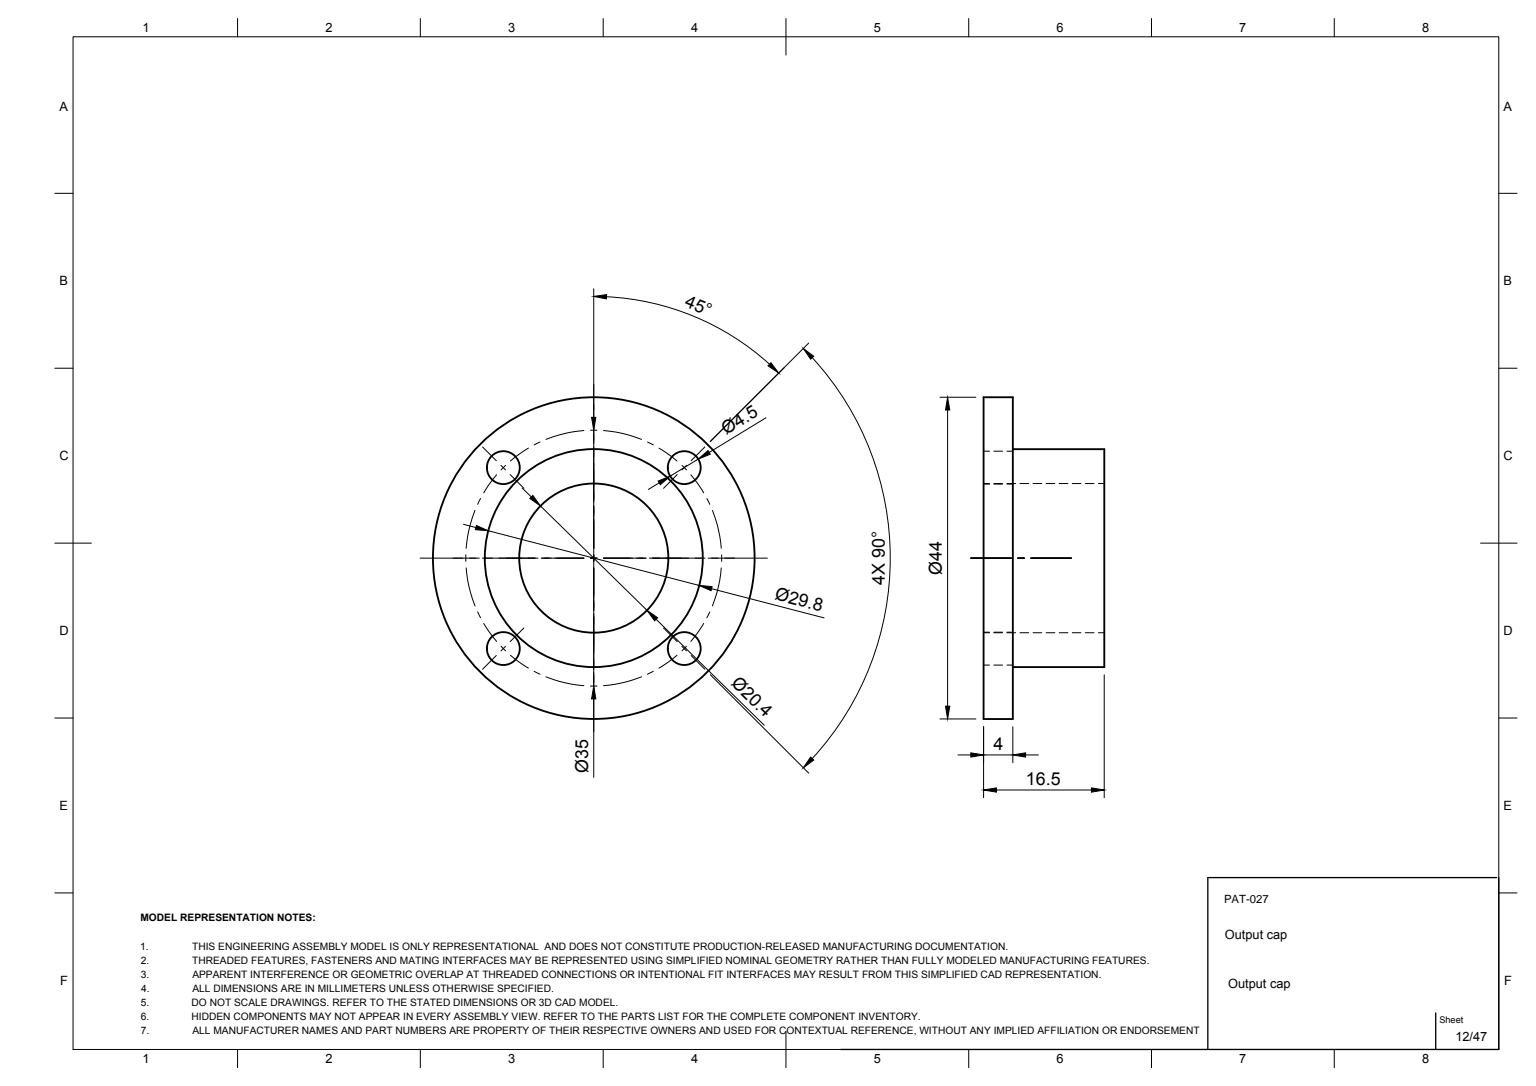
ISO-10303-21;
HEADER;
/* Generated by software containing ST-Developer
 * from STEP Tools, Inc. (www.steptools.com) 
 */

FILE_DESCRIPTION(
/* description */ ('Crank-driven oscillating fan base (mechanism only)'),

/* implementation_level */ '2;1');

FILE_NAME(
/* name */ 'Output cap.step',
/* time_stamp */ '2026-10-28T03:25:00-07:00',
/* author */ (''),
/* organization */ (''),
/* preprocessor_version */ 'ST-DEVELOPER v20.2',
/* originating_system */ 'Autodesk Translation Framework v15.17.0.0',
/* authorisation */ '');

FILE_SCHEMA (('AUTOMOTIVE_DESIGN { 1 0 10303 214 3 1 1 }'));
ENDSEC;

DATA;
#10=MECHANICAL_DESIGN_GEOMETRIC_PRESENTATION_REPRESENTATION('',(#444),#11916);
#364=SHAPE_REPRESENTATION_RELATIONSHIP('SRR','None',#12088,#404);
#404=ADVANCED_BREP_SHAPE_REPRESENTATION('',(#492),#11879);
#444=STYLED_ITEM('',(#12361),#492);
#492=MANIFOLD_SOLID_BREP('Body1',#6074);
#595=FACE_BOUND('',#1430,.T.);
#596=FACE_BOUND('',#1434,.T.);
#597=FACE_BOUND('',#1435,.T.);
#598=FACE_BOUND('',#1436,.T.);
#599=FACE_BOUND('',#1437,.T.);
#600=FACE_BOUND('',#1438,.T.);
#601=FACE_BOUND('',#1440,.T.);
#602=FACE_BOUND('',#1441,.T.);
#603=FACE_BOUND('',#1442,.T.);
#604=FACE_BOUND('',#1443,.T.);
#605=FACE_BOUND('',#1444,.T.);
#739=PLANE('',#6796);
#740=PLANE('',#6803);
#741=PLANE('',#6804);
#984=FACE_OUTER_BOUND('',#1424,.T.);
#985=FACE_OUTER_BOUND('',#1425,.T.);
#986=FACE_OUTER_BOUND('',#1426,.T.);
#987=FACE_OUTER_BOUND('',#1427,.T.);
#988=FACE_OUTER_BOUND('',#1428,.T.);
#989=FACE_OUTER_BOUND('',#1429,.T.);
#990=FACE_OUTER_BOUND('',#1431,.T.);
#991=FACE_OUTER_BOUND('',#1432,.T.);
#992=FACE_OUTER_BOUND('',#1433,.T.);
#993=FACE_OUTER_BOUND('',#1439,.T.);
#1424=EDGE_LOOP('',(#4502,#4503,#4504,#4505));
#1425=EDGE_LOOP('',(#4506,#4507,#4508,#4509));
#1426=EDGE_LOOP('',(#4510,#4511,#4512,#4513));
#1427=EDGE_LOOP('',(#4514,#4515,#4516,#4517));
#1428=EDGE_LOOP('',(#4518,#4519,#4520,#4521));
#1429=EDGE_LOOP('',(#4522));
#1430=EDGE_LOOP('',(#4523));
#1431=EDGE_LOOP('',(#4524,#4525,#4526,#4527));
#1432=EDGE_LOOP('',(#4528,#4529,#4530,#4531));
#1433=EDGE_LOOP('',(#4532));
#1434=EDGE_LOOP('',(#4533));
#1435=EDGE_LOOP('',(#4534));
#1436=EDGE_LOOP('',(#4535));
#1437=EDGE_LOOP('',(#4536));
#1438=EDGE_LOOP('',(#4537));
#1439=EDGE_LOOP('',(#4538));
#1440=EDGE_LOOP('',(#4539));
#1441=EDGE_LOOP('',(#4540));
#1442=EDGE_LOOP('',(#4541));
#1443=EDGE_LOOP('',(#4542));
#1444=EDGE_LOOP('',(#4543));
#1893=LINE('',#10059,#2226);
#1894=LINE('',#10065,#2227);
#1895=LINE('',#10071,#2228);
#1896=LINE('',#10077,#2229);
#1897=LINE('',#10083,#2230);
#1898=LINE('',#10091,#2231);
#1899=LINE('',#10096,#2232);
#2226=VECTOR('',#7954,0.225);
#2227=VECTOR('',#7961,0.225);
#2228=VECTOR('',#7968,0.225);
#2229=VECTOR('',#7975,0.225);
#2230=VECTOR('',#7982,1.49);
#2231=VECTOR('',#7993,1.02);
#2232=VECTOR('',#7998,2.2);
#2578=CIRCLE('',#6782,0.225);
#2579=CIRCLE('',#6783,0.225);
#2580=CIRCLE('',#6785,0.225);
#2581=CIRCLE('',#6786,0.225);
#2582=CIRCLE('',#6788,0.225);
#2583=CIRCLE('',#6789,0.225);
#2584=CIRCLE('',#6791,0.225);
#2585=CIRCLE('',#6792,0.225);
#2586=CIRCLE('',#6794,1.49);
#2587=CIRCLE('',#6795,1.49);
#2588=CIRCLE('',#6797,1.02);
#2589=CIRCLE('',#6799,1.02);
#2590=CIRCLE('',#6801,2.2);
#2591=CIRCLE('',#6802,2.2);
#2975=VERTEX_POINT('',#10056);
#2976=VERTEX_POINT('',#10058);
#2977=VERTEX_POINT('',#10062);
#2978=VERTEX_POINT('',#10064);
#2979=VERTEX_POINT('',#10068);
#2980=VERTEX_POINT('',#10070);
#2981=VERTEX_POINT('',#10074);
#2982=VERTEX_POINT('',#10076);
#2983=VERTEX_POINT('',#10080);
#2984=VERTEX_POINT('',#10082);
#2985=VERTEX_POINT('',#10086);
#2986=VERTEX_POINT('',#10089);
#2987=VERTEX_POINT('',#10093);
#2988=VERTEX_POINT('',#10095);
#3546=EDGE_CURVE('',#2975,#2975,#2578,.T.);
#3547=EDGE_CURVE('',#2975,#2976,#1893,.T.);
#3548=EDGE_CURVE('',#2976,#2976,#2579,.T.);
#3549=EDGE_CURVE('',#2977,#2977,#2580,.T.);
#3550=EDGE_CURVE('',#2977,#2978,#1894,.T.);
#3551=EDGE_CURVE('',#2978,#2978,#2581,.T.);
#3552=EDGE_CURVE('',#2979,#2979,#2582,.T.);
#3553=EDGE_CURVE('',#2979,#2980,#1895,.T.);
#3554=EDGE_CURVE('',#2980,#2980,#2583,.T.);
#3555=EDGE_CURVE('',#2981,#2981,#2584,.T.);
#3556=EDGE_CURVE('',#2981,#2982,#1896,.T.);
#3557=EDGE_CURVE('',#2982,#2982,#2585,.T.);
#3558=EDGE_CURVE('',#2983,#2983,#2586,.T.);
#3559=EDGE_CURVE('',#2983,#2984,#1897,.T.);
#3560=EDGE_CURVE('',#2984,#2984,#2587,.T.);
#3561=EDGE_CURVE('',#2985,#2985,#2588,.T.);
#3562=EDGE_CURVE('',#2986,#2986,#2589,.T.);
#3563=EDGE_CURVE('',#2986,#2985,#1898,.T.);
#3564=EDGE_CURVE('',#2987,#2987,#2590,.T.);
#3565=EDGE_CURVE('',#2987,#2988,#1899,.T.);
#3566=EDGE_CURVE('',#2988,#2988,#2591,.T.);
#4502=ORIENTED_EDGE('',*,*,#3546,.F.);
#4503=ORIENTED_EDGE('',*,*,#3547,.T.);
#4504=ORIENTED_EDGE('',*,*,#3548,.F.);
#4505=ORIENTED_EDGE('',*,*,#3547,.F.);
#4506=ORIENTED_EDGE('',*,*,#3549,.F.);
#4507=ORIENTED_EDGE('',*,*,#3550,.T.);
#4508=ORIENTED_EDGE('',*,*,#3551,.F.);
#4509=ORIENTED_EDGE('',*,*,#3550,.F.);
#4510=ORIENTED_EDGE('',*,*,#3552,.F.);
#4511=ORIENTED_EDGE('',*,*,#3553,.T.);
#4512=ORIENTED_EDGE('',*,*,#3554,.F.);
#4513=ORIENTED_EDGE('',*,*,#3553,.F.);
#4514=ORIENTED_EDGE('',*,*,#3555,.F.);
#4515=ORIENTED_EDGE('',*,*,#3556,.T.);
#4516=ORIENTED_EDGE('',*,*,#3557,.F.);
#4517=ORIENTED_EDGE('',*,*,#3556,.F.);
#4518=ORIENTED_EDGE('',*,*,#3558,.F.);
#4519=ORIENTED_EDGE('',*,*,#3559,.T.);
#4520=ORIENTED_EDGE('',*,*,#3560,.T.);
#4521=ORIENTED_EDGE('',*,*,#3559,.F.);
#4522=ORIENTED_EDGE('',*,*,#3560,.F.);
#4523=ORIENTED_EDGE('',*,*,#3561,.F.);
#4524=ORIENTED_EDGE('',*,*,#3562,.F.);
#4525=ORIENTED_EDGE('',*,*,#3563,.T.);
#4526=ORIENTED_EDGE('',*,*,#3561,.T.);
#4527=ORIENTED_EDGE('',*,*,#3563,.F.);
#4528=ORIENTED_EDGE('',*,*,#3564,.F.);
#4529=ORIENTED_EDGE('',*,*,#3565,.T.);
#4530=ORIENTED_EDGE('',*,*,#3566,.T.);
#4531=ORIENTED_EDGE('',*,*,#3565,.F.);
#4532=ORIENTED_EDGE('',*,*,#3564,.T.);
#4533=ORIENTED_EDGE('',*,*,#3562,.T.);
#4534=ORIENTED_EDGE('',*,*,#3557,.T.);
#4535=ORIENTED_EDGE('',*,*,#3554,.T.);
#4536=ORIENTED_EDGE('',*,*,#3551,.T.);
#4537=ORIENTED_EDGE('',*,*,#3548,.T.);
#4538=ORIENTED_EDGE('',*,*,#3566,.F.);
#4539=ORIENTED_EDGE('',*,*,#3558,.T.);
#4540=ORIENTED_EDGE('',*,*,#3555,.T.);
#4541=ORIENTED_EDGE('',*,*,#3552,.T.);
#4542=ORIENTED_EDGE('',*,*,#3549,.T.);
#4543=ORIENTED_EDGE('',*,*,#3546,.T.);
#5597=CYLINDRICAL_SURFACE('',#6781,0.225);
#5598=CYLINDRICAL_SURFACE('',#6784,0.225);
#5599=CYLINDRICAL_SURFACE('',#6787,0.225);
#5600=CYLINDRICAL_SURFACE('',#6790,0.225);
#5601=CYLINDRICAL_SURFACE('',#6793,1.49);
#5602=CYLINDRICAL_SURFACE('',#6798,1.02);
#5603=CYLINDRICAL_SURFACE('',#6800,2.2);
#5790=ADVANCED_FACE('',(#984),#5597,.F.);
#5791=ADVANCED_FACE('',(#985),#5598,.F.);
#5792=ADVANCED_FACE('',(#986),#5599,.F.);
#5793=ADVANCED_FACE('',(#987),#5600,.F.);
#5794=ADVANCED_FACE('',(#988),#5601,.T.);
#5795=ADVANCED_FACE('',(#989,#595),#739,.F.);
#5796=ADVANCED_FACE('',(#990),#5602,.F.);
#5797=ADVANCED_FACE('',(#991),#5603,.T.);
#5798=ADVANCED_FACE('',(#992,#596,#597,#598,#599,#600),#740,.T.);
#5799=ADVANCED_FACE('',(#993,#601,#602,#603,#604,#605),#741,.F.);
#6074=CLOSED_SHELL('',(#5790,#5791,#5792,#5793,#5794,#5795,#5796,#5797,
#5798,#5799));
#6780=AXIS2_PLACEMENT_3D('',#10054,#7948,#7949);
#6781=AXIS2_PLACEMENT_3D('',#10055,#7950,#7951);
#6782=AXIS2_PLACEMENT_3D('',#10057,#7952,#7953);
#6783=AXIS2_PLACEMENT_3D('',#10060,#7955,#7956);
#6784=AXIS2_PLACEMENT_3D('',#10061,#7957,#7958);
#6785=AXIS2_PLACEMENT_3D('',#10063,#7959,#7960);
#6786=AXIS2_PLACEMENT_3D('',#10066,#7962,#7963);
#6787=AXIS2_PLACEMENT_3D('',#10067,#7964,#7965);
#6788=AXIS2_PLACEMENT_3D('',#10069,#7966,#7967);
#6789=AXIS2_PLACEMENT_3D('',#10072,#7969,#7970);
#6790=AXIS2_PLACEMENT_3D('',#10073,#7971,#7972);
#6791=AXIS2_PLACEMENT_3D('',#10075,#7973,#7974);
#6792=AXIS2_PLACEMENT_3D('',#10078,#7976,#7977);
#6793=AXIS2_PLACEMENT_3D('',#10079,#7978,#7979);
#6794=AXIS2_PLACEMENT_3D('',#10081,#7980,#7981);
#6795=AXIS2_PLACEMENT_3D('',#10084,#7983,#7984);
#6796=AXIS2_PLACEMENT_3D('',#10085,#7985,#7986);
#6797=AXIS2_PLACEMENT_3D('',#10087,#7987,#7988);
#6798=AXIS2_PLACEMENT_3D('',#10088,#7989,#7990);
#6799=AXIS2_PLACEMENT_3D('',#10090,#7991,#7992);
#6800=AXIS2_PLACEMENT_3D('',#10092,#7994,#7995);
#6801=AXIS2_PLACEMENT_3D('',#10094,#7996,#7997);
#6802=AXIS2_PLACEMENT_3D('',#10097,#7999,#8000);
#6803=AXIS2_PLACEMENT_3D('',#10098,#8001,#8002);
#6804=AXIS2_PLACEMENT_3D('',#10099,#8003,#8004);
#7948=DIRECTION('axis',(0.,0.,1.));
#7949=DIRECTION('refdir',(1.,0.,0.));
#7950=DIRECTION('center_axis',(0.,0.,1.));
#7951=DIRECTION('ref_axis',(1.,0.,0.));
#7952=DIRECTION('center_axis',(0.,0.,1.));
#7953=DIRECTION('ref_axis',(1.,0.,0.));
#7954=DIRECTION('',(0.,0.,1.));
#7955=DIRECTION('center_axis',(0.,0.,-1.));
#7956=DIRECTION('ref_axis',(1.,0.,0.));
#7957=DIRECTION('center_axis',(0.,0.,1.));
#7958=DIRECTION('ref_axis',(1.,0.,0.));
#7959=DIRECTION('center_axis',(0.,0.,1.));
#7960=DIRECTION('ref_axis',(1.,0.,0.));
#7961=DIRECTION('',(0.,0.,1.));
#7962=DIRECTION('center_axis',(0.,0.,-1.));
#7963=DIRECTION('ref_axis',(1.,0.,0.));
#7964=DIRECTION('center_axis',(0.,0.,1.));
#7965=DIRECTION('ref_axis',(1.,0.,0.));
#7966=DIRECTION('center_axis',(0.,0.,1.));
#7967=DIRECTION('ref_axis',(1.,0.,0.));
#7968=DIRECTION('',(0.,0.,1.));
#7969=DIRECTION('center_axis',(0.,0.,-1.));
#7970=DIRECTION('ref_axis',(1.,0.,0.));
#7971=DIRECTION('center_axis',(0.,0.,1.));
#7972=DIRECTION('ref_axis',(1.,0.,0.));
#7973=DIRECTION('center_axis',(0.,0.,1.));
#7974=DIRECTION('ref_axis',(1.,0.,0.));
#7975=DIRECTION('',(0.,0.,1.));
#7976=DIRECTION('center_axis',(0.,0.,-1.));
#7977=DIRECTION('ref_axis',(1.,0.,0.));
#7978=DIRECTION('center_axis',(0.,0.,1.));
#7979=DIRECTION('ref_axis',(1.,0.,0.));
#7980=DIRECTION('center_axis',(0.,0.,1.));
#7981=DIRECTION('ref_axis',(1.,0.,0.));
#7982=DIRECTION('',(0.,0.,-1.));
#7983=DIRECTION('center_axis',(0.,0.,1.));
#7984=DIRECTION('ref_axis',(1.,0.,0.));
#7985=DIRECTION('center_axis',(0.,0.,1.));
#7986=DIRECTION('ref_axis',(1.,0.,0.));
#7987=DIRECTION('center_axis',(0.,0.,-1.));
#7988=DIRECTION('ref_axis',(1.,0.,0.));
#7989=DIRECTION('center_axis',(0.,0.,1.));
#7990=DIRECTION('ref_axis',(1.,0.,0.));
#7991=DIRECTION('center_axis',(0.,0.,-1.));
#7992=DIRECTION('ref_axis',(1.,0.,0.));
#7993=DIRECTION('',(0.,0.,-1.));
#7994=DIRECTION('center_axis',(0.,0.,1.));
#7995=DIRECTION('ref_axis',(1.,0.,0.));
#7996=DIRECTION('center_axis',(0.,0.,1.));
#7997=DIRECTION('ref_axis',(1.,0.,0.));
#7998=DIRECTION('',(0.,0.,-1.));
#7999=DIRECTION('center_axis',(0.,0.,1.));
#8000=DIRECTION('ref_axis',(1.,0.,0.));
#8001=DIRECTION('center_axis',(0.,0.,1.));
#8002=DIRECTION('ref_axis',(1.,0.,0.));
#8003=DIRECTION('center_axis',(0.,0.,1.));
#8004=DIRECTION('ref_axis',(1.,0.,0.));
#10054=CARTESIAN_POINT('',(0.,0.,0.));
#10055=CARTESIAN_POINT('Origin',(6.76256313292354,-1.23743686707646,5.1));
#10056=CARTESIAN_POINT('',(6.53756313292354,-1.23743686707646,5.2));
#10057=CARTESIAN_POINT('Origin',(6.76256313292354,-1.23743686707646,5.2));
#10058=CARTESIAN_POINT('',(6.53756313292354,-1.23743686707646,5.6));
#10059=CARTESIAN_POINT('',(6.53756313292354,-1.23743686707646,5.1));
#10060=CARTESIAN_POINT('Origin',(6.76256313292354,-1.23743686707646,5.6));
#10061=CARTESIAN_POINT('Origin',(6.76256313292354,1.23743686707646,5.1));
#10062=CARTESIAN_POINT('',(6.53756313292354,1.23743686707646,5.2));
#10063=CARTESIAN_POINT('Origin',(6.76256313292354,1.23743686707646,5.2));
#10064=CARTESIAN_POINT('',(6.53756313292354,1.23743686707646,5.6));
#10065=CARTESIAN_POINT('',(6.53756313292354,1.23743686707646,5.1));
#10066=CARTESIAN_POINT('Origin',(6.76256313292354,1.23743686707646,5.6));
#10067=CARTESIAN_POINT('Origin',(9.23743686707646,1.23743686707646,5.1));
#10068=CARTESIAN_POINT('',(9.01243686707646,1.23743686707646,5.2));
#10069=CARTESIAN_POINT('Origin',(9.23743686707646,1.23743686707646,5.2));
#10070=CARTESIAN_POINT('',(9.01243686707646,1.23743686707646,5.6));
#10071=CARTESIAN_POINT('',(9.01243686707646,1.23743686707646,5.1));
#10072=CARTESIAN_POINT('Origin',(9.23743686707646,1.23743686707646,5.6));
#10073=CARTESIAN_POINT('Origin',(9.23743686707646,-1.23743686707646,5.1));
#10074=CARTESIAN_POINT('',(9.01243686707646,-1.23743686707646,5.2));
#10075=CARTESIAN_POINT('Origin',(9.23743686707646,-1.23743686707646,5.2));
#10076=CARTESIAN_POINT('',(9.01243686707646,-1.23743686707646,5.6));
#10077=CARTESIAN_POINT('',(9.01243686707646,-1.23743686707646,5.1));
#10078=CARTESIAN_POINT('Origin',(9.23743686707646,-1.23743686707646,5.6));
#10079=CARTESIAN_POINT('Origin',(8.,0.,3.95));
#10080=CARTESIAN_POINT('',(6.51,-1.82472373072956E-16,5.2));
#10081=CARTESIAN_POINT('Origin',(8.,0.,5.2));
#10082=CARTESIAN_POINT('',(6.51,-1.82472373072956E-16,3.95));
#10083=CARTESIAN_POINT('',(6.51,-1.82472373072956E-16,3.95));
#10084=CARTESIAN_POINT('Origin',(8.,0.,3.95));
#10085=CARTESIAN_POINT('Origin',(8.,0.,3.95));
#10086=CARTESIAN_POINT('',(6.98,-1.2491397351303E-16,3.95));
#10087=CARTESIAN_POINT('Origin',(8.,0.,3.95));
#10088=CARTESIAN_POINT('Origin',(8.,0.,5.2));
#10089=CARTESIAN_POINT('',(6.98,-1.2491397351303E-16,5.6));
#10090=CARTESIAN_POINT('Origin',(8.,0.,5.6));
#10091=CARTESIAN_POINT('',(6.98,-1.2491397351303E-16,5.2));
#10092=CARTESIAN_POINT('Origin',(8.,0.,5.2));
#10093=CARTESIAN_POINT('',(5.8,-2.69422295812418E-16,5.6));
#10094=CARTESIAN_POINT('Origin',(8.,0.,5.6));
#10095=CARTESIAN_POINT('',(5.8,-2.69422295812418E-16,5.2));
#10096=CARTESIAN_POINT('',(5.8,-2.69422295812418E-16,5.2));
#10097=CARTESIAN_POINT('Origin',(8.,0.,5.2));
#10098=CARTESIAN_POINT('Origin',(8.,0.,5.6));
#10099=CARTESIAN_POINT('Origin',(8.,0.,5.2));
#11832=UNCERTAINTY_MEASURE_WITH_UNIT(LENGTH_MEASURE(0.001),#11917,
'DISTANCE_ACCURACY_VALUE',
'Maximum model space distance between geometric entities at asserted c
onnectivities');
#11869=UNCERTAINTY_MEASURE_WITH_UNIT(LENGTH_MEASURE(0.001),#11917,
'DISTANCE_ACCURACY_VALUE',
'Maximum model space distance between geometric entities at asserted c
onnectivities');
#11879=(
GEOMETRIC_REPRESENTATION_CONTEXT(3)
GLOBAL_UNCERTAINTY_ASSIGNED_CONTEXT((#11832))
GLOBAL_UNIT_ASSIGNED_CONTEXT((#11917,#11919,#11920))
REPRESENTATION_CONTEXT('','3D')
);
#11916=(
GEOMETRIC_REPRESENTATION_CONTEXT(3)
GLOBAL_UNCERTAINTY_ASSIGNED_CONTEXT((#11869))
GLOBAL_UNIT_ASSIGNED_CONTEXT((#11917,#11919,#11920))
REPRESENTATION_CONTEXT('','3D')
);
#11917=(
LENGTH_UNIT()
NAMED_UNIT(*)
SI_UNIT(.CENTI.,.METRE.)
);
#11919=(
NAMED_UNIT(*)
PLANE_ANGLE_UNIT()
SI_UNIT($,.RADIAN.)
);
#11920=(
NAMED_UNIT(*)
SI_UNIT($,.STERADIAN.)
SOLID_ANGLE_UNIT()
);
#11930=SHAPE_DEFINITION_REPRESENTATION(#11976,#12088);
#11976=PRODUCT_DEFINITION_SHAPE('',$,#12135);
#12088=SHAPE_REPRESENTATION('',(#6780),#11879);
#12125=PRODUCT_DEFINITION_CONTEXT('part definition',#12265,'design');
#12135=PRODUCT_DEFINITION('Output cap','Output cap',#12181,#12125);
#12181=PRODUCT_DEFINITION_FORMATION('',$,#12276);
#12265=APPLICATION_CONTEXT(
'Core Data for Automotive Mechanical Design Process');
#12266=PRODUCT_CONTEXT('part definition',#12265,'mechanical');
#12276=PRODUCT('Output cap','Output cap','Output cap',(#12266));
#12355=COLOUR_RGB('Light Blue',0.38,0.62,0.78);
#12356=FILL_AREA_STYLE_COLOUR('',#12355);
#12357=FILL_AREA_STYLE('',(#12356));
#12358=SURFACE_STYLE_FILL_AREA(#12357);
#12359=SURFACE_SIDE_STYLE('',(#12358));
#12360=SURFACE_STYLE_USAGE(.BOTH.,#12359);
#12361=PRESENTATION_STYLE_ASSIGNMENT((#12360));
ENDSEC;
END-ISO-10303-21;
